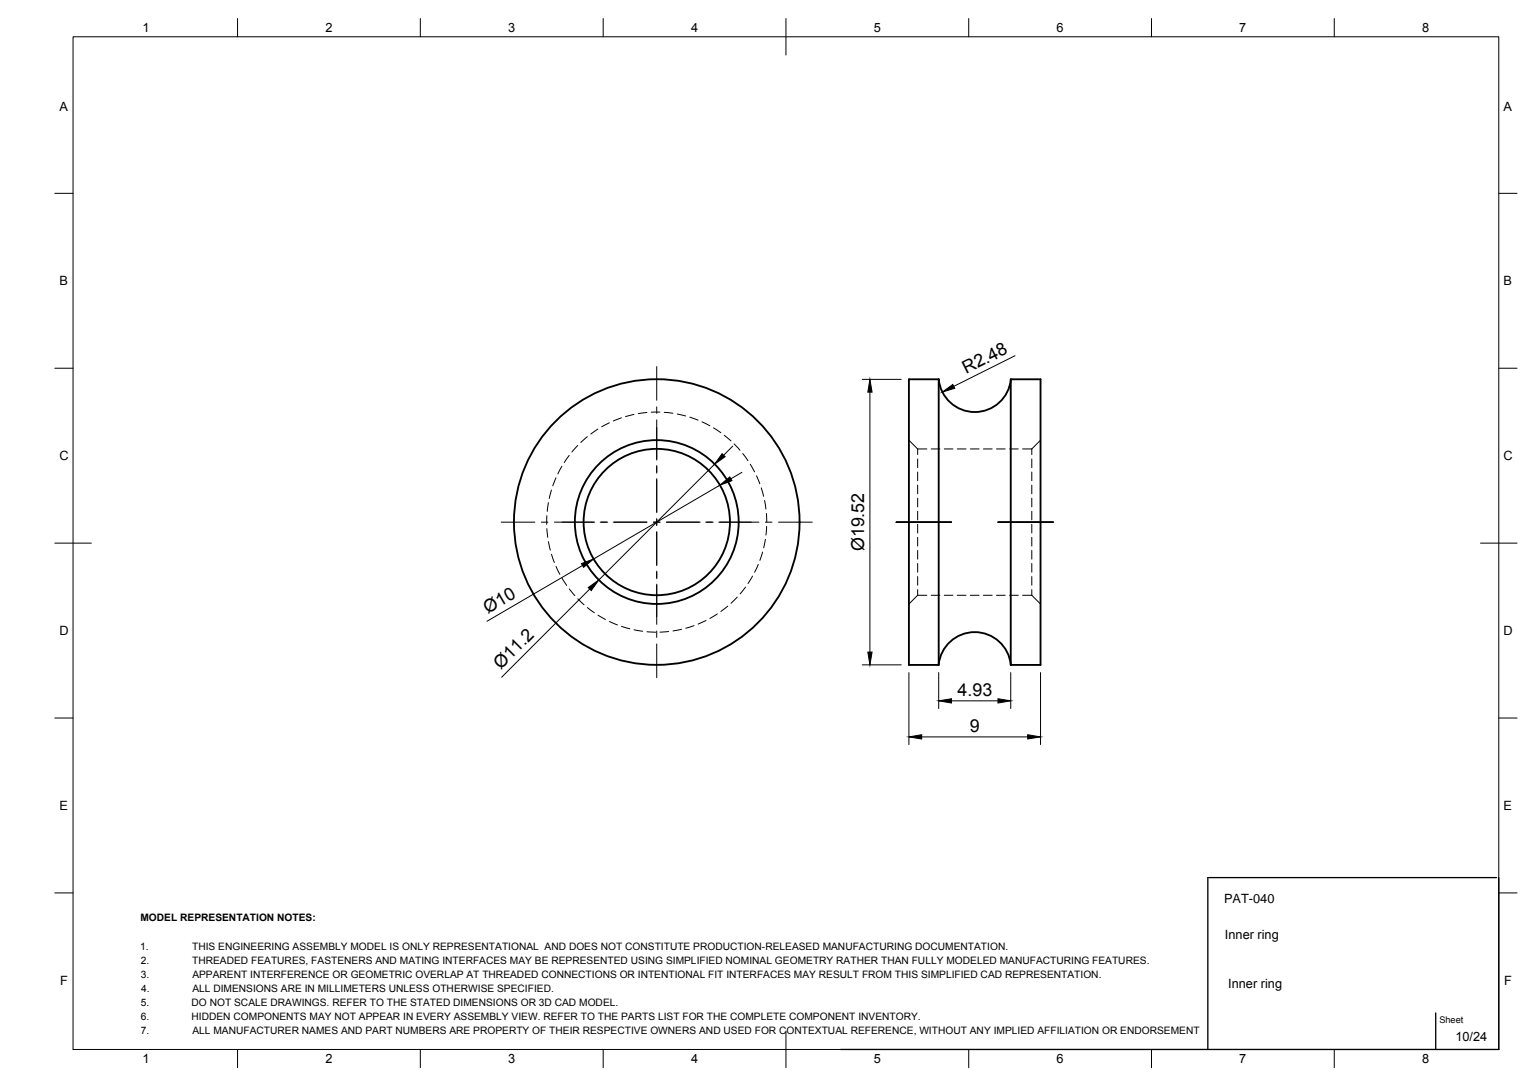
ISO-10303-21;
HEADER;
/* Generated by software containing ST-Developer
 * from STEP Tools, Inc. (www.steptools.com) 
 */

FILE_DESCRIPTION(
/* description */ ('Four-bar tabletop demonstrator'),
/* implementation_level */ '2;1');

FILE_NAME(
/* name */ 'Inner ring.step',
/* time_stamp */ '2026-10-29T17:05:23-07:00',
/* author */ (''),
/* organization */ (''),
/* preprocessor_version */ 'ST-DEVELOPER v20.2',
/* originating_system */ 'Autodesk Translation Framework v15.17.0.0',
/* authorisation */ '');

FILE_SCHEMA (('AUTOMOTIVE_DESIGN { 1 0 10303 214 3 1 1 }'));
ENDSEC;

DATA;
#10=MECHANICAL_DESIGN_GEOMETRIC_PRESENTATION_REPRESENTATION('',(#341),#6705);
#263=TOROIDAL_SURFACE('',#3749,1.,0.247676);
#268=CONICAL_SURFACE('',#3760,0.53,0.785398163397448);
#269=CONICAL_SURFACE('',#3767,0.53,0.785398163397448);
#311=SHAPE_REPRESENTATION_RELATIONSHIP('SRR','None',#6820,#326);
#326=ADVANCED_BREP_SHAPE_REPRESENTATION('',(#363),#6693);
#341=STYLED_ITEM('',(#6989),#363);
#363=MANIFOLD_SOLID_BREP('Body1',#3386);
#426=FACE_BOUND('',#897,.T.);
#427=FACE_BOUND('',#900,.T.);
#504=PLANE('',#3762);
#505=PLANE('',#3765);
#644=FACE_OUTER_BOUND('',#892,.T.);
#645=FACE_OUTER_BOUND('',#893,.T.);
#646=FACE_OUTER_BOUND('',#894,.T.);
#647=FACE_OUTER_BOUND('',#895,.T.);
#648=FACE_OUTER_BOUND('',#896,.T.);
#649=FACE_OUTER_BOUND('',#898,.T.);
#650=FACE_OUTER_BOUND('',#899,.T.);
#651=FACE_OUTER_BOUND('',#901,.T.);
#892=EDGE_LOOP('',(#2628,#2629,#2630,#2631,#2632,#2633));
#893=EDGE_LOOP('',(#2634,#2635,#2636,#2637,#2638));
#894=EDGE_LOOP('',(#2639,#2640,#2641,#2642));
#895=EDGE_LOOP('',(#2643,#2644,#2645,#2646));
#896=EDGE_LOOP('',(#2647));
#897=EDGE_LOOP('',(#2648));
#898=EDGE_LOOP('',(#2649,#2650,#2651,#2652,#2653));
#899=EDGE_LOOP('',(#2654));
#900=EDGE_LOOP('',(#2655));
#901=EDGE_LOOP('',(#2656,#2657,#2658,#2659));
#1130=LINE('',#5679,#1300);
#1131=LINE('',#5685,#1301);
#1132=LINE('',#5689,#1302);
#1133=LINE('',#5695,#1303);
#1134=LINE('',#5700,#1304);
#1300=VECTOR('',#4515,0.976185);
#1301=VECTOR('',#4522,0.5);
#1302=VECTOR('',#4527,0.53);
#1303=VECTOR('',#4536,0.976185);
#1304=VECTOR('',#4543,0.53);
#1474=CIRCLE('',#3750,0.976185);
#1475=CIRCLE('',#3751,0.976185);
#1476=CIRCLE('',#3752,0.247676);
#1477=CIRCLE('',#3753,0.976185);
#1478=CIRCLE('',#3754,0.976185);
#1479=CIRCLE('',#3756,0.976185);
#1480=CIRCLE('',#3758,0.5);
#1481=CIRCLE('',#3759,0.5);
#1482=CIRCLE('',#3761,0.56);
#1483=CIRCLE('',#3764,0.976185);
#1484=CIRCLE('',#3766,0.56);
#1713=VERTEX_POINT('',#5668);
#1714=VERTEX_POINT('',#5669);
#1715=VERTEX_POINT('',#5672);
#1716=VERTEX_POINT('',#5674);
#1717=VERTEX_POINT('',#5678);
#1718=VERTEX_POINT('',#5682);
#1719=VERTEX_POINT('',#5684);
#1720=VERTEX_POINT('',#5688);
#1721=VERTEX_POINT('',#5693);
#1722=VERTEX_POINT('',#5697);
#2050=EDGE_CURVE('',#1713,#1714,#1474,.T.);
#2051=EDGE_CURVE('',#1714,#1713,#1475,.T.);
#2052=EDGE_CURVE('',#1714,#1715,#1476,.T.);
#2053=EDGE_CURVE('',#1716,#1715,#1477,.T.);
#2054=EDGE_CURVE('',#1715,#1716,#1478,.T.);
#2055=EDGE_CURVE('',#1716,#1717,#1130,.T.);
#2056=EDGE_CURVE('',#1717,#1717,#1479,.T.);
#2057=EDGE_CURVE('',#1718,#1718,#1480,.T.);
#2058=EDGE_CURVE('',#1718,#1719,#1131,.T.);
#2059=EDGE_CURVE('',#1719,#1719,#1481,.T.);
#2060=EDGE_CURVE('',#1719,#1720,#1132,.T.);
#2061=EDGE_CURVE('',#1720,#1720,#1482,.T.);
#2062=EDGE_CURVE('',#1721,#1721,#1483,.T.);
#2063=EDGE_CURVE('',#1721,#1713,#1133,.T.);
#2064=EDGE_CURVE('',#1722,#1722,#1484,.T.);
#2065=EDGE_CURVE('',#1722,#1718,#1134,.T.);
#2628=ORIENTED_EDGE('',*,*,#2050,.F.);
#2629=ORIENTED_EDGE('',*,*,#2051,.F.);
#2630=ORIENTED_EDGE('',*,*,#2052,.T.);
#2631=ORIENTED_EDGE('',*,*,#2053,.F.);
#2632=ORIENTED_EDGE('',*,*,#2054,.F.);
#2633=ORIENTED_EDGE('',*,*,#2052,.F.);
#2634=ORIENTED_EDGE('',*,*,#2053,.T.);
#2635=ORIENTED_EDGE('',*,*,#2054,.T.);
#2636=ORIENTED_EDGE('',*,*,#2055,.T.);
#2637=ORIENTED_EDGE('',*,*,#2056,.T.);
#2638=ORIENTED_EDGE('',*,*,#2055,.F.);
#2639=ORIENTED_EDGE('',*,*,#2057,.T.);
#2640=ORIENTED_EDGE('',*,*,#2058,.T.);
#2641=ORIENTED_EDGE('',*,*,#2059,.F.);
#2642=ORIENTED_EDGE('',*,*,#2058,.F.);
#2643=ORIENTED_EDGE('',*,*,#2059,.T.);
#2644=ORIENTED_EDGE('',*,*,#2060,.T.);
#2645=ORIENTED_EDGE('',*,*,#2061,.F.);
#2646=ORIENTED_EDGE('',*,*,#2060,.F.);
#2647=ORIENTED_EDGE('',*,*,#2056,.F.);
#2648=ORIENTED_EDGE('',*,*,#2061,.T.);
#2649=ORIENTED_EDGE('',*,*,#2062,.F.);
#2650=ORIENTED_EDGE('',*,*,#2063,.T.);
#2651=ORIENTED_EDGE('',*,*,#2050,.T.);
#2652=ORIENTED_EDGE('',*,*,#2051,.T.);
#2653=ORIENTED_EDGE('',*,*,#2063,.F.);
#2654=ORIENTED_EDGE('',*,*,#2062,.T.);
#2655=ORIENTED_EDGE('',*,*,#2064,.F.);
#2656=ORIENTED_EDGE('',*,*,#2064,.T.);
#2657=ORIENTED_EDGE('',*,*,#2065,.T.);
#2658=ORIENTED_EDGE('',*,*,#2057,.F.);
#2659=ORIENTED_EDGE('',*,*,#2065,.F.);
#3141=CYLINDRICAL_SURFACE('',#3755,0.976185);
#3142=CYLINDRICAL_SURFACE('',#3757,0.5);
#3143=CYLINDRICAL_SURFACE('',#3763,0.976185);
#3260=ADVANCED_FACE('',(#644),#263,.F.);
#3261=ADVANCED_FACE('',(#645),#3141,.T.);
#3262=ADVANCED_FACE('',(#646),#3142,.F.);
#3263=ADVANCED_FACE('',(#647),#268,.F.);
#3264=ADVANCED_FACE('',(#648,#426),#504,.T.);
#3265=ADVANCED_FACE('',(#649),#3143,.T.);
#3266=ADVANCED_FACE('',(#650,#427),#505,.T.);
#3267=ADVANCED_FACE('',(#651),#269,.F.);
#3386=CLOSED_SHELL('',(#3260,#3261,#3262,#3263,#3264,#3265,#3266,#3267));
#3748=AXIS2_PLACEMENT_3D('',#5666,#4499,#4500);
#3749=AXIS2_PLACEMENT_3D('',#5667,#4501,#4502);
#3750=AXIS2_PLACEMENT_3D('',#5670,#4503,#4504);
#3751=AXIS2_PLACEMENT_3D('',#5671,#4505,#4506);
#3752=AXIS2_PLACEMENT_3D('',#5673,#4507,#4508);
#3753=AXIS2_PLACEMENT_3D('',#5675,#4509,#4510);
#3754=AXIS2_PLACEMENT_3D('',#5676,#4511,#4512);
#3755=AXIS2_PLACEMENT_3D('',#5677,#4513,#4514);
#3756=AXIS2_PLACEMENT_3D('',#5680,#4516,#4517);
#3757=AXIS2_PLACEMENT_3D('',#5681,#4518,#4519);
#3758=AXIS2_PLACEMENT_3D('',#5683,#4520,#4521);
#3759=AXIS2_PLACEMENT_3D('',#5686,#4523,#4524);
#3760=AXIS2_PLACEMENT_3D('',#5687,#4525,#4526);
#3761=AXIS2_PLACEMENT_3D('',#5690,#4528,#4529);
#3762=AXIS2_PLACEMENT_3D('',#5691,#4530,#4531);
#3763=AXIS2_PLACEMENT_3D('',#5692,#4532,#4533);
#3764=AXIS2_PLACEMENT_3D('',#5694,#4534,#4535);
#3765=AXIS2_PLACEMENT_3D('',#5696,#4537,#4538);
#3766=AXIS2_PLACEMENT_3D('',#5698,#4539,#4540);
#3767=AXIS2_PLACEMENT_3D('',#5699,#4541,#4542);
#4499=DIRECTION('axis',(0.,0.,1.));
#4500=DIRECTION('refdir',(1.,0.,0.));
#4501=DIRECTION('center_axis',(0.,-1.,0.));
#4502=DIRECTION('ref_axis',(0.,0.,-1.));
#4503=DIRECTION('center_axis',(0.,-1.,0.));
#4504=DIRECTION('ref_axis',(1.,0.,0.));
#4505=DIRECTION('center_axis',(0.,-1.,0.));
#4506=DIRECTION('ref_axis',(1.,0.,0.));
#4507=DIRECTION('center_axis',(1.,0.,1.22464679914735E-16));
#4508=DIRECTION('ref_axis',(-1.22464679914735E-16,0.,1.));
#4509=DIRECTION('center_axis',(0.,1.,0.));
#4510=DIRECTION('ref_axis',(1.,0.,0.));
#4511=DIRECTION('center_axis',(0.,1.,0.));
#4512=DIRECTION('ref_axis',(1.,0.,0.));
#4513=DIRECTION('center_axis',(0.,-1.,0.));
#4514=DIRECTION('ref_axis',(1.,0.,0.));
#4515=DIRECTION('',(0.,1.,0.));
#4516=DIRECTION('center_axis',(0.,-1.,0.));
#4517=DIRECTION('ref_axis',(1.,0.,0.));
#4518=DIRECTION('center_axis',(0.,-1.,0.));
#4519=DIRECTION('ref_axis',(1.,0.,0.));
#4520=DIRECTION('center_axis',(0.,-1.,0.));
#4521=DIRECTION('ref_axis',(1.,0.,0.));
#4522=DIRECTION('',(0.,1.,0.));
#4523=DIRECTION('center_axis',(0.,-1.,0.));
#4524=DIRECTION('ref_axis',(1.,0.,0.));
#4525=DIRECTION('center_axis',(0.,1.,0.));
#4526=DIRECTION('ref_axis',(1.,0.,0.));
#4527=DIRECTION('',(-0.707106781186547,0.707106781186548,-8.65956056235493E-17));
#4528=DIRECTION('center_axis',(0.,-1.,0.));
#4529=DIRECTION('ref_axis',(1.,0.,0.));
#4530=DIRECTION('center_axis',(0.,1.,0.));
#4531=DIRECTION('ref_axis',(0.,0.,1.));
#4532=DIRECTION('center_axis',(0.,-1.,0.));
#4533=DIRECTION('ref_axis',(1.,0.,0.));
#4534=DIRECTION('center_axis',(0.,-1.,0.));
#4535=DIRECTION('ref_axis',(1.,0.,0.));
#4536=DIRECTION('',(0.,1.,0.));
#4537=DIRECTION('center_axis',(0.,-1.,0.));
#4538=DIRECTION('ref_axis',(0.,0.,-1.));
#4539=DIRECTION('center_axis',(0.,-1.,0.));
#4540=DIRECTION('ref_axis',(1.,0.,0.));
#4541=DIRECTION('center_axis',(0.,-1.,0.));
#4542=DIRECTION('ref_axis',(1.,0.,0.));
#4543=DIRECTION('',(0.707106781186547,0.707106781186548,8.65956056235493E-17));
#5666=CARTESIAN_POINT('',(0.,0.,0.));
#5667=CARTESIAN_POINT('Origin',(0.,0.,0.));
#5668=CARTESIAN_POINT('',(-0.976185,-0.246528389340863,-1.19548183562566E-16));
#5669=CARTESIAN_POINT('',(-1.19548183562566E-16,-0.246528389340863,0.976185));
#5670=CARTESIAN_POINT('Origin',(0.,-0.246528389340863,0.));
#5671=CARTESIAN_POINT('Origin',(0.,-0.246528389340863,0.));
#5672=CARTESIAN_POINT('',(-1.19548183562566E-16,0.246528389340863,0.976185));
#5673=CARTESIAN_POINT('Origin',(-1.22464679914735E-16,0.,1.));
#5674=CARTESIAN_POINT('',(-0.976185,0.246528389340863,1.19548183562566E-16));
#5675=CARTESIAN_POINT('Origin',(0.,0.246528389340863,0.));
#5676=CARTESIAN_POINT('Origin',(0.,0.246528389340863,0.));
#5677=CARTESIAN_POINT('Origin',(0.,0.,0.));
#5678=CARTESIAN_POINT('',(-0.976185,0.45,-1.19548183562566E-16));
#5679=CARTESIAN_POINT('',(-0.976185,0.,-1.19548183562566E-16));
#5680=CARTESIAN_POINT('Origin',(0.,0.45,0.));
#5681=CARTESIAN_POINT('Origin',(0.,0.,0.));
#5682=CARTESIAN_POINT('',(-0.5,-0.39,-6.12323399573677E-17));
#5683=CARTESIAN_POINT('Origin',(0.,-0.39,0.));
#5684=CARTESIAN_POINT('',(-0.5,0.39,-6.12323399573677E-17));
#5685=CARTESIAN_POINT('',(-0.5,0.,-6.12323399573677E-17));
#5686=CARTESIAN_POINT('Origin',(0.,0.39,0.));
#5687=CARTESIAN_POINT('Origin',(0.,0.42,0.));
#5688=CARTESIAN_POINT('',(-0.56,0.45,-6.85802207522518E-17));
#5689=CARTESIAN_POINT('',(-0.53,0.42,-6.49062803548097E-17));
#5690=CARTESIAN_POINT('Origin',(0.,0.45,0.));
#5691=CARTESIAN_POINT('Origin',(0.976185,0.45,0.));
#5692=CARTESIAN_POINT('Origin',(0.,0.,0.));
#5693=CARTESIAN_POINT('',(-0.976185,-0.45,-1.19548183562566E-16));
#5694=CARTESIAN_POINT('Origin',(0.,-0.45,0.));
#5695=CARTESIAN_POINT('',(-0.976185,0.,-1.19548183562566E-16));
#5696=CARTESIAN_POINT('Origin',(0.56,-0.45,0.));
#5697=CARTESIAN_POINT('',(-0.56,-0.45,-6.85802207522518E-17));
#5698=CARTESIAN_POINT('Origin',(0.,-0.45,0.));
#5699=CARTESIAN_POINT('Origin',(0.,-0.42,0.));
#5700=CARTESIAN_POINT('',(-0.53,-0.42,-6.49062803548097E-17));
#6671=UNCERTAINTY_MEASURE_WITH_UNIT(LENGTH_MEASURE(0.001),#6706,
'DISTANCE_ACCURACY_VALUE',
'Maximum model space distance between geometric entities at asserted c
onnectivities');
#6683=UNCERTAINTY_MEASURE_WITH_UNIT(LENGTH_MEASURE(0.001),#6706,
'DISTANCE_ACCURACY_VALUE',
'Maximum model space distance between geometric entities at asserted c
onnectivities');
#6693=(
GEOMETRIC_REPRESENTATION_CONTEXT(3)
GLOBAL_UNCERTAINTY_ASSIGNED_CONTEXT((#6671))
GLOBAL_UNIT_ASSIGNED_CONTEXT((#6706,#6708,#6709))
REPRESENTATION_CONTEXT('','3D')
);
#6705=(
GEOMETRIC_REPRESENTATION_CONTEXT(3)
GLOBAL_UNCERTAINTY_ASSIGNED_CONTEXT((#6683))
GLOBAL_UNIT_ASSIGNED_CONTEXT((#6706,#6708,#6709))
REPRESENTATION_CONTEXT('','3D')
);
#6706=(
LENGTH_UNIT()
NAMED_UNIT(*)
SI_UNIT(.CENTI.,.METRE.)
);
#6708=(
NAMED_UNIT(*)
PLANE_ANGLE_UNIT()
SI_UNIT($,.RADIAN.)
);
#6709=(
NAMED_UNIT(*)
SI_UNIT($,.STERADIAN.)
SOLID_ANGLE_UNIT()
);
#6719=SHAPE_DEFINITION_REPRESENTATION(#6740,#6820);
#6740=PRODUCT_DEFINITION_SHAPE('',$,#6842);
#6820=SHAPE_REPRESENTATION('',(#3748),#6693);
#6832=PRODUCT_DEFINITION_CONTEXT('part definition',#6897,'design');
#6842=PRODUCT_DEFINITION('Inner ring','Inner ring',#6863,#6832);
#6863=PRODUCT_DEFINITION_FORMATION('',$,#6908);
#6897=APPLICATION_CONTEXT(
'Core Data for Automotive Mechanical Design Process');
#6898=PRODUCT_CONTEXT('part definition',#6897,'mechanical');
#6908=PRODUCT('Inner ring','Inner ring','Inner ring',(#6898));
#6983=COLOUR_RGB('Grey',0.48,0.52,0.57);
#6984=FILL_AREA_STYLE_COLOUR('',#6983);
#6985=FILL_AREA_STYLE('',(#6984));
#6986=SURFACE_STYLE_FILL_AREA(#6985);
#6987=SURFACE_SIDE_STYLE('',(#6986));
#6988=SURFACE_STYLE_USAGE(.BOTH.,#6987);
#6989=PRESENTATION_STYLE_ASSIGNMENT((#6988));
ENDSEC;
END-ISO-10303-21;
